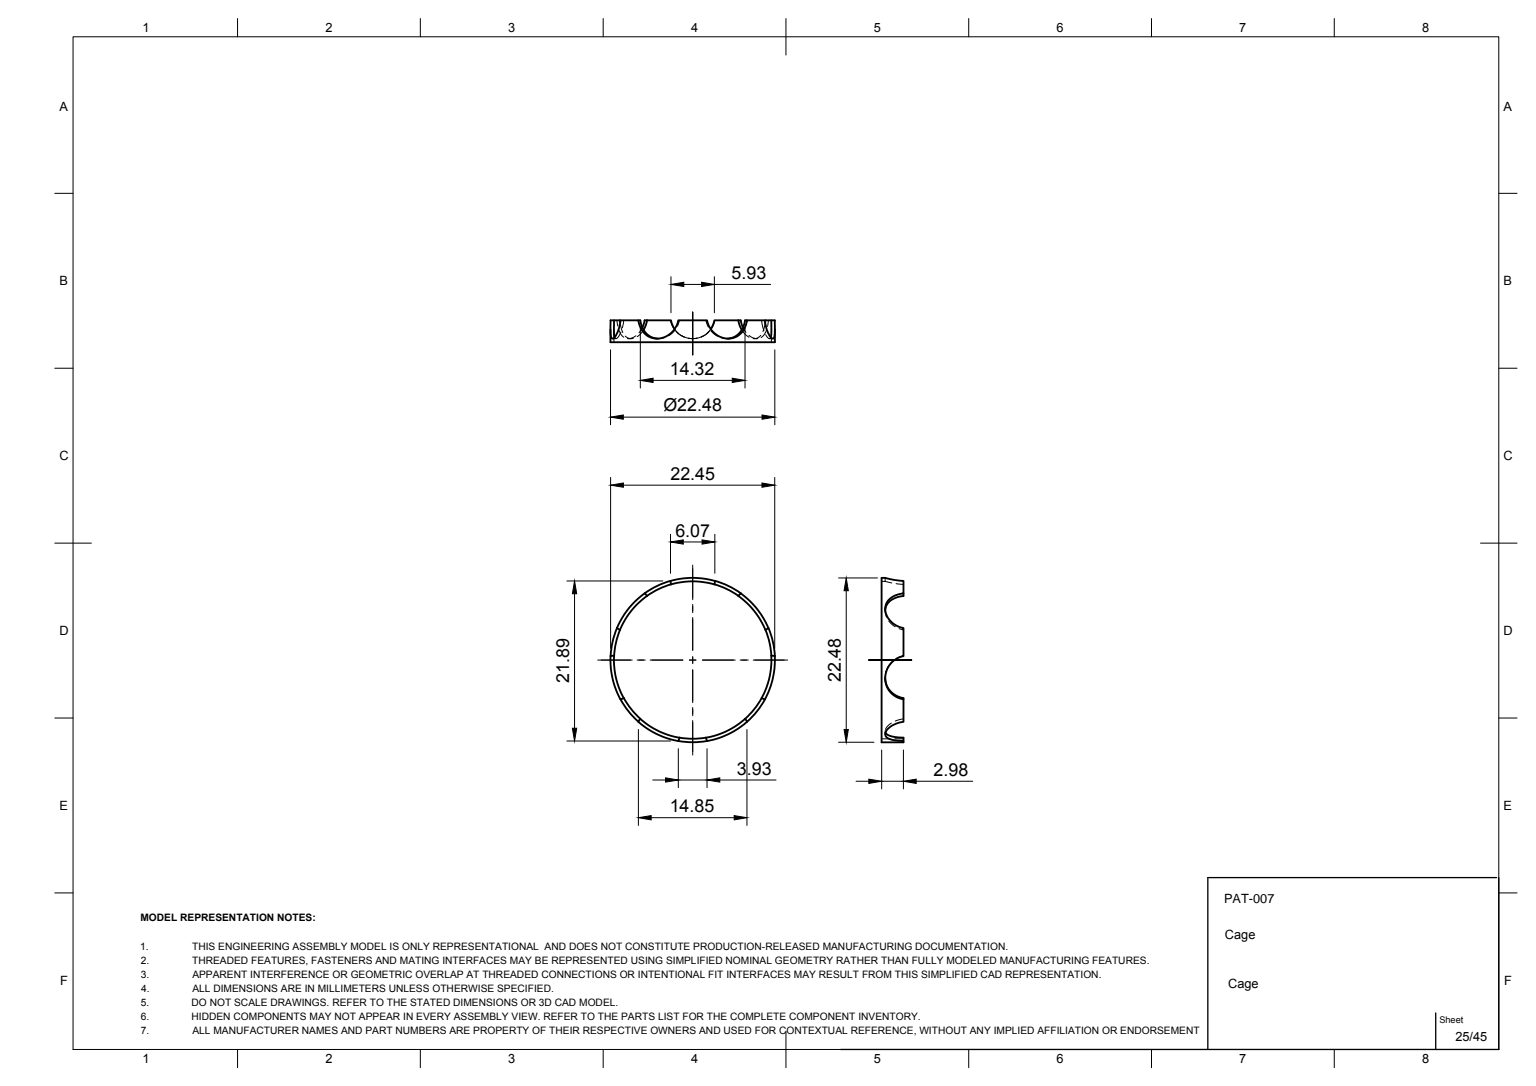
ISO-10303-21;
HEADER;
/* Generated by software containing ST-Developer
 * from STEP Tools, Inc. (www.steptools.com) 
 */

FILE_DESCRIPTION(
/* description */ ('Bearing friction torque test rig'),
/* implementation_level */ '2;1');

FILE_NAME(
/* name */ 'Cage.step',
/* time_stamp */ '2026-10-28T03:24:04-07:00',
/* author */ (''),
/* organization */ (''),
/* preprocessor_version */ 'ST-DEVELOPER v20.2',
/* originating_system */ 'Autodesk Translation Framework v15.17.0.0',
/* authorisation */ '');

FILE_SCHEMA (('AUTOMOTIVE_DESIGN { 1 0 10303 214 3 1 1 }'));
ENDSEC;

DATA;
#10=MECHANICAL_DESIGN_GEOMETRIC_PRESENTATION_REPRESENTATION('',(#564),#14822);
#343=B_SPLINE_CURVE_WITH_KNOTS('',3,(#12896,#12897,#12898,#12899,#12900,
#12901,#12902,#12903,#12904,#12905,#12906,#12907,#12908,#12909,#12910,#12911,
#12912,#12913,#12914,#12915,#12916,#12917),.UNSPECIFIED.,.F.,.F.,(4,2,2,
2,2,2,2,2,2,2,4),(0.0591825211272536,0.157966726598481,0.236950089897721,
0.315933453196962,0.391576304923761,0.46721915665056,0.54286200837736,0.618504860104159,
0.697488223403399,0.77647158670264,0.875255792173867),.UNSPECIFIED.);
#344=B_SPLINE_CURVE_WITH_KNOTS('',3,(#12921,#12922,#12923,#12924,#12925,
#12926,#12927,#12928,#12929,#12930,#12931,#12932,#12933,#12934,#12935,#12936,
#12937,#12938,#12939,#12940,#12941,#12942),.UNSPECIFIED.,.F.,.F.,(4,2,2,
2,2,2,2,2,2,2,4),(0.0581119756758434,0.106553146291161,0.213106292582322,
0.30849933801665,0.386091982889075,0.4636846277615,0.541277272633925,0.61886991750635,
0.714262962940678,0.820816109231839,0.869257279847157),.UNSPECIFIED.);
#345=B_SPLINE_CURVE_WITH_KNOTS('',3,(#12948,#12949,#12950,#12951,#12952,
#12953,#12954,#12955,#12956,#12957,#12958,#12959,#12960,#12961,#12962,#12963,
#12964,#12965,#12966,#12967,#12968,#12969),.UNSPECIFIED.,.F.,.F.,(4,2,2,
2,2,2,2,2,2,2,4),(0.0581119756758434,0.106553146291161,0.213106292582322,
0.30849933801665,0.386091982889075,0.4636846277615,0.541277272633925,0.61886991750635,
0.714262962940679,0.820816109231839,0.869257279847157),.UNSPECIFIED.);
#346=B_SPLINE_CURVE_WITH_KNOTS('',3,(#12973,#12974,#12975,#12976,#12977,
#12978,#12979,#12980,#12981,#12982,#12983,#12984,#12985,#12986,#12987,#12988,
#12989,#12990,#12991,#12992,#12993,#12994),.UNSPECIFIED.,.F.,.F.,(4,2,2,
2,2,2,2,2,2,2,4),(0.0581119756758433,0.106553146291161,0.213106292582322,
0.308499338016649,0.386091982889075,0.4636846277615,0.541277272633925,0.61886991750635,
0.714262962940678,0.820816109231839,0.869257279847157),.UNSPECIFIED.);
#347=B_SPLINE_CURVE_WITH_KNOTS('',3,(#13003,#13004,#13005,#13006,#13007,
#13008,#13009,#13010,#13011,#13012,#13013,#13014,#13015,#13016,#13017,#13018,
#13019,#13020,#13021,#13022,#13023,#13024),.UNSPECIFIED.,.F.,.F.,(4,2,2,
2,2,2,2,2,2,2,4),(0.0581119756758433,0.106553146291161,0.213106292582322,
0.30849933801665,0.386091982889075,0.4636846277615,0.541277272633925,0.61886991750635,
0.714262962940678,0.820816109231839,0.869257279847157),.UNSPECIFIED.);
#348=B_SPLINE_CURVE_WITH_KNOTS('',3,(#13028,#13029,#13030,#13031,#13032,
#13033,#13034,#13035,#13036,#13037,#13038,#13039,#13040,#13041,#13042,#13043,
#13044,#13045,#13046,#13047,#13048,#13049),.UNSPECIFIED.,.F.,.F.,(4,2,2,
2,2,2,2,2,2,2,4),(0.0581119756758434,0.106553146291161,0.213106292582322,
0.30849933801665,0.386091982889075,0.4636846277615,0.541277272633925,0.61886991750635,
0.714262962940678,0.820816109231839,0.869257279847157),.UNSPECIFIED.);
#349=B_SPLINE_CURVE_WITH_KNOTS('',3,(#13053,#13054,#13055,#13056,#13057,
#13058,#13059,#13060,#13061,#13062,#13063,#13064,#13065,#13066,#13067,#13068,
#13069,#13070,#13071,#13072,#13073,#13074),.UNSPECIFIED.,.F.,.F.,(4,2,2,
2,2,2,2,2,2,2,4),(0.0581119756758434,0.106553146291161,0.213106292582322,
0.30849933801665,0.386091982889075,0.4636846277615,0.541277272633925,0.61886991750635,
0.714262962940678,0.820816109231839,0.869257279847157),.UNSPECIFIED.);
#350=B_SPLINE_CURVE_WITH_KNOTS('',3,(#13078,#13079,#13080,#13081,#13082,
#13083,#13084,#13085,#13086,#13087,#13088,#13089,#13090,#13091,#13092,#13093,
#13094,#13095,#13096,#13097,#13098,#13099),.UNSPECIFIED.,.F.,.F.,(4,2,2,
2,2,2,2,2,2,2,4),(0.0581119756758433,0.106553146291161,0.213106292582322,
0.30849933801665,0.386091982889075,0.4636846277615,0.541277272633925,0.61886991750635,
0.714262962940678,0.820816109231839,0.869257279847157),.UNSPECIFIED.);
#351=B_SPLINE_CURVE_WITH_KNOTS('',3,(#13107,#13108,#13109,#13110,#13111,
#13112,#13113,#13114,#13115,#13116,#13117,#13118,#13119,#13120,#13121,#13122,
#13123,#13124,#13125,#13126,#13127,#13128),.UNSPECIFIED.,.F.,.F.,(4,2,2,
2,2,2,2,2,2,2,4),(0.0591825211272536,0.157966726598481,0.236950089897721,
0.315933453196962,0.391576304923761,0.467219156650561,0.54286200837736,
0.618504860104159,0.697488223403399,0.77647158670264,0.875255792173867),
 .UNSPECIFIED.);
#352=B_SPLINE_CURVE_WITH_KNOTS('',3,(#13136,#13137,#13138,#13139,#13140,
#13141,#13142,#13143,#13144,#13145,#13146,#13147,#13148,#13149,#13150,#13151,
#13152,#13153,#13154,#13155,#13156,#13157),.UNSPECIFIED.,.F.,.F.,(4,2,2,
2,2,2,2,2,2,2,4),(0.0591825211272536,0.157966726598481,0.236950089897722,
0.315933453196962,0.391576304923761,0.467219156650561,0.54286200837736,
0.618504860104159,0.697488223403399,0.77647158670264,0.875255792173867),
 .UNSPECIFIED.);
#353=B_SPLINE_CURVE_WITH_KNOTS('',3,(#13167,#13168,#13169,#13170,#13171,
#13172,#13173,#13174,#13175,#13176,#13177,#13178,#13179,#13180,#13181,#13182,
#13183,#13184,#13185,#13186,#13187,#13188),.UNSPECIFIED.,.F.,.F.,(4,2,2,
2,2,2,2,2,2,2,4),(0.0591825211272536,0.157966726598481,0.236950089897721,
0.315933453196962,0.391576304923761,0.46721915665056,0.54286200837736,0.618504860104159,
0.697488223403399,0.77647158670264,0.875255792173867),.UNSPECIFIED.);
#354=B_SPLINE_CURVE_WITH_KNOTS('',3,(#13196,#13197,#13198,#13199,#13200,
#13201,#13202,#13203,#13204,#13205,#13206,#13207,#13208,#13209,#13210,#13211,
#13212,#13213,#13214,#13215,#13216,#13217),.UNSPECIFIED.,.F.,.F.,(4,2,2,
2,2,2,2,2,2,2,4),(0.0591825211272536,0.157966726598481,0.236950089897721,
0.315933453196962,0.391576304923761,0.46721915665056,0.542862008377359,
0.618504860104159,0.697488223403399,0.776471586702639,0.875255792173867),
 .UNSPECIFIED.);
#355=B_SPLINE_CURVE_WITH_KNOTS('',3,(#13225,#13226,#13227,#13228,#13229,
#13230,#13231,#13232,#13233,#13234,#13235,#13236,#13237,#13238,#13239,#13240,
#13241,#13242,#13243,#13244,#13245,#13246),.UNSPECIFIED.,.F.,.F.,(4,2,2,
2,2,2,2,2,2,2,4),(0.0591825211272536,0.157966726598481,0.236950089897721,
0.315933453196962,0.391576304923761,0.46721915665056,0.54286200837736,0.618504860104159,
0.697488223403399,0.77647158670264,0.875255792173867),.UNSPECIFIED.);
#356=B_SPLINE_CURVE_WITH_KNOTS('',3,(#13255,#13256,#13257,#13258,#13259,
#13260,#13261,#13262,#13263,#13264,#13265,#13266,#13267,#13268,#13269,#13270,
#13271,#13272,#13273,#13274,#13275,#13276),.UNSPECIFIED.,.F.,.F.,(4,2,2,
2,2,2,2,2,2,2,4),(0.0591825211272536,0.157966726598481,0.236950089897721,
0.315933453196962,0.391576304923761,0.46721915665056,0.542862008377359,
0.618504860104159,0.697488223403399,0.776471586702639,0.875255792173867),
 .UNSPECIFIED.);
#402=SPHERICAL_SURFACE('',#8679,0.309556);
#403=SPHERICAL_SURFACE('',#8695,0.309556);
#404=SPHERICAL_SURFACE('',#8700,0.309556);
#405=SPHERICAL_SURFACE('',#8706,0.309556);
#406=SPHERICAL_SURFACE('',#8711,0.309556);
#407=SPHERICAL_SURFACE('',#8716,0.309556);
#408=SPHERICAL_SURFACE('',#8724,0.309556);
#480=SHAPE_REPRESENTATION_RELATIONSHIP('SRR','None',#15020,#519);
#519=ADVANCED_BREP_SHAPE_REPRESENTATION('',(#617),#14800);
#564=STYLED_ITEM('',(#15284),#617);
#617=MANIFOLD_SOLID_BREP('Continuous crown cage',#7681);
#818=FACE_BOUND('',#1994,.T.);
#1006=PLANE('',#8692);
#1007=PLANE('',#8697);
#1008=PLANE('',#8702);
#1009=PLANE('',#8708);
#1010=PLANE('',#8713);
#1011=PLANE('',#8722);
#1012=PLANE('',#8726);
#1013=PLANE('',#8727);
#1359=FACE_OUTER_BOUND('',#1978,.T.);
#1360=FACE_OUTER_BOUND('',#1979,.T.);
#1361=FACE_OUTER_BOUND('',#1980,.T.);
#1362=FACE_OUTER_BOUND('',#1981,.T.);
#1363=FACE_OUTER_BOUND('',#1982,.T.);
#1364=FACE_OUTER_BOUND('',#1983,.T.);
#1365=FACE_OUTER_BOUND('',#1984,.T.);
#1366=FACE_OUTER_BOUND('',#1985,.T.);
#1367=FACE_OUTER_BOUND('',#1986,.T.);
#1368=FACE_OUTER_BOUND('',#1987,.T.);
#1369=FACE_OUTER_BOUND('',#1988,.T.);
#1370=FACE_OUTER_BOUND('',#1989,.T.);
#1371=FACE_OUTER_BOUND('',#1990,.T.);
#1372=FACE_OUTER_BOUND('',#1991,.T.);
#1373=FACE_OUTER_BOUND('',#1992,.T.);
#1374=FACE_OUTER_BOUND('',#1993,.T.);
#1375=FACE_OUTER_BOUND('',#1995,.T.);
#1978=EDGE_LOOP('',(#6282,#6283,#6284,#6285));
#1979=EDGE_LOOP('',(#6286,#6287,#6288,#6289,#6290,#6291,#6292,#6293,#6294,
#6295,#6296,#6297,#6298,#6299,#6300,#6301,#6302,#6303));
#1980=EDGE_LOOP('',(#6304,#6305,#6306,#6307));
#1981=EDGE_LOOP('',(#6308,#6309,#6310,#6311));
#1982=EDGE_LOOP('',(#6312,#6313,#6314,#6315));
#1983=EDGE_LOOP('',(#6316,#6317,#6318,#6319));
#1984=EDGE_LOOP('',(#6320,#6321,#6322,#6323,#6324,#6325));
#1985=EDGE_LOOP('',(#6326,#6327,#6328,#6329));
#1986=EDGE_LOOP('',(#6330,#6331,#6332,#6333));
#1987=EDGE_LOOP('',(#6334,#6335,#6336,#6337));
#1988=EDGE_LOOP('',(#6338,#6339,#6340,#6341));
#1989=EDGE_LOOP('',(#6342,#6343,#6344,#6345));
#1990=EDGE_LOOP('',(#6346,#6347,#6348,#6349,#6350,#6351,#6352,#6353,#6354,
#6355,#6356,#6357,#6358,#6359,#6360,#6361,#6362,#6363));
#1991=EDGE_LOOP('',(#6364,#6365,#6366,#6367));
#1992=EDGE_LOOP('',(#6368,#6369,#6370,#6371));
#1993=EDGE_LOOP('',(#6372));
#1994=EDGE_LOOP('',(#6373));
#1995=EDGE_LOOP('',(#6374,#6375,#6376,#6377));
#2532=LINE('',#12998,#2976);
#2533=LINE('',#13251,#2977);
#2976=VECTOR('',#10567,1.123812);
#2977=VECTOR('',#10636,1.076188);
#3355=CIRCLE('',#8680,0.303778037777585);
#3356=CIRCLE('',#8681,0.303778037777585);
#3357=CIRCLE('',#8683,1.123812);
#3358=CIRCLE('',#8684,1.123812);
#3359=CIRCLE('',#8685,1.123812);
#3360=CIRCLE('',#8686,1.123812);
#3361=CIRCLE('',#8687,1.123812);
#3362=CIRCLE('',#8688,1.123812);
#3363=CIRCLE('',#8689,1.123812);
#3364=CIRCLE('',#8690,1.123812);
#3365=CIRCLE('',#8691,1.123812);
#3366=CIRCLE('',#8693,1.076188);
#3367=CIRCLE('',#8694,0.303778037777585);
#3368=CIRCLE('',#8696,0.303778037777585);
#3369=CIRCLE('',#8698,1.076188);
#3370=CIRCLE('',#8699,0.303778037777585);
#3371=CIRCLE('',#8701,0.303778037777585);
#3372=CIRCLE('',#8703,1.076188);
#3373=CIRCLE('',#8704,1.076188);
#3374=CIRCLE('',#8705,0.303778037777585);
#3375=CIRCLE('',#8707,0.303778037777585);
#3376=CIRCLE('',#8709,1.076188);
#3377=CIRCLE('',#8710,0.303778037777585);
#3378=CIRCLE('',#8712,0.303778037777585);
#3379=CIRCLE('',#8714,1.076188);
#3380=CIRCLE('',#8715,0.303778037777585);
#3381=CIRCLE('',#8717,0.303778037777585);
#3382=CIRCLE('',#8719,1.076188);
#3383=CIRCLE('',#8720,1.076188);
#3384=CIRCLE('',#8721,1.076188);
#3385=CIRCLE('',#8723,0.303778037777585);
#3386=CIRCLE('',#8725,0.303778037777585);
#3938=VERTEX_POINT('',#12894);
#3939=VERTEX_POINT('',#12895);
#3940=VERTEX_POINT('',#12918);
#3941=VERTEX_POINT('',#12920);
#3942=VERTEX_POINT('',#12945);
#3943=VERTEX_POINT('',#12947);
#3944=VERTEX_POINT('',#12970);
#3945=VERTEX_POINT('',#12972);
#3946=VERTEX_POINT('',#12995);
#3947=VERTEX_POINT('',#12997);
#3948=VERTEX_POINT('',#13000);
#3949=VERTEX_POINT('',#13002);
#3950=VERTEX_POINT('',#13025);
#3951=VERTEX_POINT('',#13027);
#3952=VERTEX_POINT('',#13050);
#3953=VERTEX_POINT('',#13052);
#3954=VERTEX_POINT('',#13075);
#3955=VERTEX_POINT('',#13077);
#3956=VERTEX_POINT('',#13102);
#3957=VERTEX_POINT('',#13106);
#3958=VERTEX_POINT('',#13131);
#3959=VERTEX_POINT('',#13135);
#3960=VERTEX_POINT('',#13160);
#3961=VERTEX_POINT('',#13162);
#3962=VERTEX_POINT('',#13166);
#3963=VERTEX_POINT('',#13191);
#3964=VERTEX_POINT('',#13195);
#3965=VERTEX_POINT('',#13220);
#3966=VERTEX_POINT('',#13224);
#3967=VERTEX_POINT('',#13249);
#3968=VERTEX_POINT('',#13252);
#3969=VERTEX_POINT('',#13254);
#4767=EDGE_CURVE('',#3938,#3939,#343,.T.);
#4768=EDGE_CURVE('',#3940,#3938,#3355,.T.);
#4769=EDGE_CURVE('',#3941,#3940,#344,.T.);
#4770=EDGE_CURVE('',#3939,#3941,#3356,.T.);
#4771=EDGE_CURVE('',#3942,#3940,#3357,.T.);
#4772=EDGE_CURVE('',#3942,#3943,#345,.T.);
#4773=EDGE_CURVE('',#3944,#3943,#3358,.T.);
#4774=EDGE_CURVE('',#3944,#3945,#346,.T.);
#4775=EDGE_CURVE('',#3946,#3945,#3359,.T.);
#4776=EDGE_CURVE('',#3946,#3947,#2532,.T.);
#4777=EDGE_CURVE('',#3947,#3947,#3360,.T.);
#4778=EDGE_CURVE('',#3948,#3946,#3361,.T.);
#4779=EDGE_CURVE('',#3948,#3949,#347,.T.);
#4780=EDGE_CURVE('',#3950,#3949,#3362,.T.);
#4781=EDGE_CURVE('',#3950,#3951,#348,.T.);
#4782=EDGE_CURVE('',#3952,#3951,#3363,.T.);
#4783=EDGE_CURVE('',#3952,#3953,#349,.T.);
#4784=EDGE_CURVE('',#3954,#3953,#3364,.T.);
#4785=EDGE_CURVE('',#3954,#3955,#350,.T.);
#4786=EDGE_CURVE('',#3941,#3955,#3365,.T.);
#4787=EDGE_CURVE('',#3938,#3956,#3366,.T.);
#4788=EDGE_CURVE('',#3956,#3942,#3367,.T.);
#4789=EDGE_CURVE('',#3957,#3956,#351,.T.);
#4790=EDGE_CURVE('',#3943,#3957,#3368,.T.);
#4791=EDGE_CURVE('',#3957,#3958,#3369,.T.);
#4792=EDGE_CURVE('',#3958,#3944,#3370,.T.);
#4793=EDGE_CURVE('',#3959,#3958,#352,.T.);
#4794=EDGE_CURVE('',#3945,#3959,#3371,.T.);
#4795=EDGE_CURVE('',#3959,#3960,#3372,.T.);
#4796=EDGE_CURVE('',#3960,#3961,#3373,.T.);
#4797=EDGE_CURVE('',#3961,#3948,#3374,.T.);
#4798=EDGE_CURVE('',#3962,#3961,#353,.T.);
#4799=EDGE_CURVE('',#3949,#3962,#3375,.T.);
#4800=EDGE_CURVE('',#3962,#3963,#3376,.T.);
#4801=EDGE_CURVE('',#3963,#3950,#3377,.T.);
#4802=EDGE_CURVE('',#3964,#3963,#354,.T.);
#4803=EDGE_CURVE('',#3951,#3964,#3378,.T.);
#4804=EDGE_CURVE('',#3964,#3965,#3379,.T.);
#4805=EDGE_CURVE('',#3965,#3952,#3380,.T.);
#4806=EDGE_CURVE('',#3966,#3965,#355,.T.);
#4807=EDGE_CURVE('',#3953,#3966,#3381,.T.);
#4808=EDGE_CURVE('',#3967,#3967,#3382,.T.);
#4809=EDGE_CURVE('',#3967,#3960,#2533,.T.);
#4810=EDGE_CURVE('',#3968,#3939,#3383,.T.);
#4811=EDGE_CURVE('',#3968,#3969,#356,.T.);
#4812=EDGE_CURVE('',#3966,#3969,#3384,.T.);
#4813=EDGE_CURVE('',#3955,#3968,#3385,.T.);
#4814=EDGE_CURVE('',#3969,#3954,#3386,.T.);
#6282=ORIENTED_EDGE('',*,*,#4767,.F.);
#6283=ORIENTED_EDGE('',*,*,#4768,.F.);
#6284=ORIENTED_EDGE('',*,*,#4769,.F.);
#6285=ORIENTED_EDGE('',*,*,#4770,.F.);
#6286=ORIENTED_EDGE('',*,*,#4769,.T.);
#6287=ORIENTED_EDGE('',*,*,#4771,.F.);
#6288=ORIENTED_EDGE('',*,*,#4772,.T.);
#6289=ORIENTED_EDGE('',*,*,#4773,.F.);
#6290=ORIENTED_EDGE('',*,*,#4774,.T.);
#6291=ORIENTED_EDGE('',*,*,#4775,.F.);
#6292=ORIENTED_EDGE('',*,*,#4776,.T.);
#6293=ORIENTED_EDGE('',*,*,#4777,.F.);
#6294=ORIENTED_EDGE('',*,*,#4776,.F.);
#6295=ORIENTED_EDGE('',*,*,#4778,.F.);
#6296=ORIENTED_EDGE('',*,*,#4779,.T.);
#6297=ORIENTED_EDGE('',*,*,#4780,.F.);
#6298=ORIENTED_EDGE('',*,*,#4781,.T.);
#6299=ORIENTED_EDGE('',*,*,#4782,.F.);
#6300=ORIENTED_EDGE('',*,*,#4783,.T.);
#6301=ORIENTED_EDGE('',*,*,#4784,.F.);
#6302=ORIENTED_EDGE('',*,*,#4785,.T.);
#6303=ORIENTED_EDGE('',*,*,#4786,.F.);
#6304=ORIENTED_EDGE('',*,*,#4768,.T.);
#6305=ORIENTED_EDGE('',*,*,#4787,.T.);
#6306=ORIENTED_EDGE('',*,*,#4788,.T.);
#6307=ORIENTED_EDGE('',*,*,#4771,.T.);
#6308=ORIENTED_EDGE('',*,*,#4789,.F.);
#6309=ORIENTED_EDGE('',*,*,#4790,.F.);
#6310=ORIENTED_EDGE('',*,*,#4772,.F.);
#6311=ORIENTED_EDGE('',*,*,#4788,.F.);
#6312=ORIENTED_EDGE('',*,*,#4790,.T.);
#6313=ORIENTED_EDGE('',*,*,#4791,.T.);
#6314=ORIENTED_EDGE('',*,*,#4792,.T.);
#6315=ORIENTED_EDGE('',*,*,#4773,.T.);
#6316=ORIENTED_EDGE('',*,*,#4793,.F.);
#6317=ORIENTED_EDGE('',*,*,#4794,.F.);
#6318=ORIENTED_EDGE('',*,*,#4774,.F.);
#6319=ORIENTED_EDGE('',*,*,#4792,.F.);
#6320=ORIENTED_EDGE('',*,*,#4794,.T.);
#6321=ORIENTED_EDGE('',*,*,#4795,.T.);
#6322=ORIENTED_EDGE('',*,*,#4796,.T.);
#6323=ORIENTED_EDGE('',*,*,#4797,.T.);
#6324=ORIENTED_EDGE('',*,*,#4778,.T.);
#6325=ORIENTED_EDGE('',*,*,#4775,.T.);
#6326=ORIENTED_EDGE('',*,*,#4798,.F.);
#6327=ORIENTED_EDGE('',*,*,#4799,.F.);
#6328=ORIENTED_EDGE('',*,*,#4779,.F.);
#6329=ORIENTED_EDGE('',*,*,#4797,.F.);
#6330=ORIENTED_EDGE('',*,*,#4799,.T.);
#6331=ORIENTED_EDGE('',*,*,#4800,.T.);
#6332=ORIENTED_EDGE('',*,*,#4801,.T.);
#6333=ORIENTED_EDGE('',*,*,#4780,.T.);
#6334=ORIENTED_EDGE('',*,*,#4802,.F.);
#6335=ORIENTED_EDGE('',*,*,#4803,.F.);
#6336=ORIENTED_EDGE('',*,*,#4781,.F.);
#6337=ORIENTED_EDGE('',*,*,#4801,.F.);
#6338=ORIENTED_EDGE('',*,*,#4803,.T.);
#6339=ORIENTED_EDGE('',*,*,#4804,.T.);
#6340=ORIENTED_EDGE('',*,*,#4805,.T.);
#6341=ORIENTED_EDGE('',*,*,#4782,.T.);
#6342=ORIENTED_EDGE('',*,*,#4783,.F.);
#6343=ORIENTED_EDGE('',*,*,#4805,.F.);
#6344=ORIENTED_EDGE('',*,*,#4806,.F.);
#6345=ORIENTED_EDGE('',*,*,#4807,.F.);
#6346=ORIENTED_EDGE('',*,*,#4808,.F.);
#6347=ORIENTED_EDGE('',*,*,#4809,.T.);
#6348=ORIENTED_EDGE('',*,*,#4795,.F.);
#6349=ORIENTED_EDGE('',*,*,#4793,.T.);
#6350=ORIENTED_EDGE('',*,*,#4791,.F.);
#6351=ORIENTED_EDGE('',*,*,#4789,.T.);
#6352=ORIENTED_EDGE('',*,*,#4787,.F.);
#6353=ORIENTED_EDGE('',*,*,#4767,.T.);
#6354=ORIENTED_EDGE('',*,*,#4810,.F.);
#6355=ORIENTED_EDGE('',*,*,#4811,.T.);
#6356=ORIENTED_EDGE('',*,*,#4812,.F.);
#6357=ORIENTED_EDGE('',*,*,#4806,.T.);
#6358=ORIENTED_EDGE('',*,*,#4804,.F.);
#6359=ORIENTED_EDGE('',*,*,#4802,.T.);
#6360=ORIENTED_EDGE('',*,*,#4800,.F.);
#6361=ORIENTED_EDGE('',*,*,#4798,.T.);
#6362=ORIENTED_EDGE('',*,*,#4796,.F.);
#6363=ORIENTED_EDGE('',*,*,#4809,.F.);
#6364=ORIENTED_EDGE('',*,*,#4770,.T.);
#6365=ORIENTED_EDGE('',*,*,#4786,.T.);
#6366=ORIENTED_EDGE('',*,*,#4813,.T.);
#6367=ORIENTED_EDGE('',*,*,#4810,.T.);
#6368=ORIENTED_EDGE('',*,*,#4785,.F.);
#6369=ORIENTED_EDGE('',*,*,#4814,.F.);
#6370=ORIENTED_EDGE('',*,*,#4811,.F.);
#6371=ORIENTED_EDGE('',*,*,#4813,.F.);
#6372=ORIENTED_EDGE('',*,*,#4777,.T.);
#6373=ORIENTED_EDGE('',*,*,#4808,.T.);
#6374=ORIENTED_EDGE('',*,*,#4807,.T.);
#6375=ORIENTED_EDGE('',*,*,#4812,.T.);
#6376=ORIENTED_EDGE('',*,*,#4814,.T.);
#6377=ORIENTED_EDGE('',*,*,#4784,.T.);
#7156=CYLINDRICAL_SURFACE('',#8682,1.123812);
#7157=CYLINDRICAL_SURFACE('',#8718,1.076188);
#7470=ADVANCED_FACE('',(#1359),#402,.F.);
#7471=ADVANCED_FACE('',(#1360),#7156,.T.);
#7472=ADVANCED_FACE('',(#1361),#1006,.T.);
#7473=ADVANCED_FACE('',(#1362),#403,.F.);
#7474=ADVANCED_FACE('',(#1363),#1007,.T.);
#7475=ADVANCED_FACE('',(#1364),#404,.F.);
#7476=ADVANCED_FACE('',(#1365),#1008,.T.);
#7477=ADVANCED_FACE('',(#1366),#405,.F.);
#7478=ADVANCED_FACE('',(#1367),#1009,.T.);
#7479=ADVANCED_FACE('',(#1368),#406,.F.);
#7480=ADVANCED_FACE('',(#1369),#1010,.T.);
#7481=ADVANCED_FACE('',(#1370),#407,.F.);
#7482=ADVANCED_FACE('',(#1371),#7157,.F.);
#7483=ADVANCED_FACE('',(#1372),#1011,.T.);
#7484=ADVANCED_FACE('',(#1373),#408,.F.);
#7485=ADVANCED_FACE('',(#1374,#818),#1012,.T.);
#7486=ADVANCED_FACE('',(#1375),#1013,.T.);
#7681=CLOSED_SHELL('',(#7470,#7471,#7472,#7473,#7474,#7475,#7476,#7477,
#7478,#7479,#7480,#7481,#7482,#7483,#7484,#7485,#7486));
#8678=AXIS2_PLACEMENT_3D('',#12892,#10551,#10552);
#8679=AXIS2_PLACEMENT_3D('',#12893,#10553,#10554);
#8680=AXIS2_PLACEMENT_3D('',#12919,#10555,#10556);
#8681=AXIS2_PLACEMENT_3D('',#12943,#10557,#10558);
#8682=AXIS2_PLACEMENT_3D('',#12944,#10559,#10560);
#8683=AXIS2_PLACEMENT_3D('',#12946,#10561,#10562);
#8684=AXIS2_PLACEMENT_3D('',#12971,#10563,#10564);
#8685=AXIS2_PLACEMENT_3D('',#12996,#10565,#10566);
#8686=AXIS2_PLACEMENT_3D('',#12999,#10568,#10569);
#8687=AXIS2_PLACEMENT_3D('',#13001,#10570,#10571);
#8688=AXIS2_PLACEMENT_3D('',#13026,#10572,#10573);
#8689=AXIS2_PLACEMENT_3D('',#13051,#10574,#10575);
#8690=AXIS2_PLACEMENT_3D('',#13076,#10576,#10577);
#8691=AXIS2_PLACEMENT_3D('',#13100,#10578,#10579);
#8692=AXIS2_PLACEMENT_3D('',#13101,#10580,#10581);
#8693=AXIS2_PLACEMENT_3D('',#13103,#10582,#10583);
#8694=AXIS2_PLACEMENT_3D('',#13104,#10584,#10585);
#8695=AXIS2_PLACEMENT_3D('',#13105,#10586,#10587);
#8696=AXIS2_PLACEMENT_3D('',#13129,#10588,#10589);
#8697=AXIS2_PLACEMENT_3D('',#13130,#10590,#10591);
#8698=AXIS2_PLACEMENT_3D('',#13132,#10592,#10593);
#8699=AXIS2_PLACEMENT_3D('',#13133,#10594,#10595);
#8700=AXIS2_PLACEMENT_3D('',#13134,#10596,#10597);
#8701=AXIS2_PLACEMENT_3D('',#13158,#10598,#10599);
#8702=AXIS2_PLACEMENT_3D('',#13159,#10600,#10601);
#8703=AXIS2_PLACEMENT_3D('',#13161,#10602,#10603);
#8704=AXIS2_PLACEMENT_3D('',#13163,#10604,#10605);
#8705=AXIS2_PLACEMENT_3D('',#13164,#10606,#10607);
#8706=AXIS2_PLACEMENT_3D('',#13165,#10608,#10609);
#8707=AXIS2_PLACEMENT_3D('',#13189,#10610,#10611);
#8708=AXIS2_PLACEMENT_3D('',#13190,#10612,#10613);
#8709=AXIS2_PLACEMENT_3D('',#13192,#10614,#10615);
#8710=AXIS2_PLACEMENT_3D('',#13193,#10616,#10617);
#8711=AXIS2_PLACEMENT_3D('',#13194,#10618,#10619);
#8712=AXIS2_PLACEMENT_3D('',#13218,#10620,#10621);
#8713=AXIS2_PLACEMENT_3D('',#13219,#10622,#10623);
#8714=AXIS2_PLACEMENT_3D('',#13221,#10624,#10625);
#8715=AXIS2_PLACEMENT_3D('',#13222,#10626,#10627);
#8716=AXIS2_PLACEMENT_3D('',#13223,#10628,#10629);
#8717=AXIS2_PLACEMENT_3D('',#13247,#10630,#10631);
#8718=AXIS2_PLACEMENT_3D('',#13248,#10632,#10633);
#8719=AXIS2_PLACEMENT_3D('',#13250,#10634,#10635);
#8720=AXIS2_PLACEMENT_3D('',#13253,#10637,#10638);
#8721=AXIS2_PLACEMENT_3D('',#13277,#10639,#10640);
#8722=AXIS2_PLACEMENT_3D('',#13278,#10641,#10642);
#8723=AXIS2_PLACEMENT_3D('',#13279,#10643,#10644);
#8724=AXIS2_PLACEMENT_3D('',#13280,#10645,#10646);
#8725=AXIS2_PLACEMENT_3D('',#13281,#10647,#10648);
#8726=AXIS2_PLACEMENT_3D('',#13282,#10649,#10650);
#8727=AXIS2_PLACEMENT_3D('',#13283,#10651,#10652);
#10551=DIRECTION('axis',(0.,0.,1.));
#10552=DIRECTION('refdir',(1.,0.,0.));
#10553=DIRECTION('center_axis',(0.,0.,1.));
#10554=DIRECTION('ref_axis',(1.,0.,0.));
#10555=DIRECTION('center_axis',(0.,-1.,0.));
#10556=DIRECTION('ref_axis',(0.,0.,-1.));
#10557=DIRECTION('center_axis',(0.,-1.,0.));
#10558=DIRECTION('ref_axis',(0.,0.,-1.));
#10559=DIRECTION('center_axis',(0.,1.,0.));
#10560=DIRECTION('ref_axis',(1.,0.,0.));
#10561=DIRECTION('center_axis',(0.,1.,0.));
#10562=DIRECTION('ref_axis',(1.,0.,0.));
#10563=DIRECTION('center_axis',(0.,1.,0.));
#10564=DIRECTION('ref_axis',(1.,0.,0.));
#10565=DIRECTION('center_axis',(0.,1.,0.));
#10566=DIRECTION('ref_axis',(1.,0.,0.));
#10567=DIRECTION('',(0.,-1.,0.));
#10568=DIRECTION('center_axis',(0.,-1.,0.));
#10569=DIRECTION('ref_axis',(1.,0.,0.));
#10570=DIRECTION('center_axis',(0.,1.,0.));
#10571=DIRECTION('ref_axis',(1.,0.,0.));
#10572=DIRECTION('center_axis',(0.,1.,0.));
#10573=DIRECTION('ref_axis',(1.,0.,0.));
#10574=DIRECTION('center_axis',(0.,1.,0.));
#10575=DIRECTION('ref_axis',(1.,0.,0.));
#10576=DIRECTION('center_axis',(0.,1.,0.));
#10577=DIRECTION('ref_axis',(1.,0.,0.));
#10578=DIRECTION('center_axis',(0.,1.,0.));
#10579=DIRECTION('ref_axis',(1.,0.,0.));
#10580=DIRECTION('center_axis',(0.,1.,0.));
#10581=DIRECTION('ref_axis',(1.,0.,0.));
#10582=DIRECTION('center_axis',(0.,-1.,0.));
#10583=DIRECTION('ref_axis',(1.,0.,0.));
#10584=DIRECTION('center_axis',(0.,-1.,0.));
#10585=DIRECTION('ref_axis',(0.,0.,-1.));
#10586=DIRECTION('center_axis',(8.96625347776458E-17,0.,1.));
#10587=DIRECTION('ref_axis',(1.,0.,0.));
#10588=DIRECTION('center_axis',(0.,-1.,0.));
#10589=DIRECTION('ref_axis',(0.,0.,-1.));
#10590=DIRECTION('center_axis',(0.,1.,0.));
#10591=DIRECTION('ref_axis',(1.,0.,0.));
#10592=DIRECTION('center_axis',(0.,-1.,0.));
#10593=DIRECTION('ref_axis',(1.,0.,0.));
#10594=DIRECTION('center_axis',(0.,-1.,0.));
#10595=DIRECTION('ref_axis',(0.,0.,-1.));
#10596=DIRECTION('center_axis',(0.,0.,1.));
#10597=DIRECTION('ref_axis',(1.,0.,0.));
#10598=DIRECTION('center_axis',(0.,-1.,0.));
#10599=DIRECTION('ref_axis',(0.,0.,-1.));
#10600=DIRECTION('center_axis',(0.,1.,0.));
#10601=DIRECTION('ref_axis',(1.,0.,0.));
#10602=DIRECTION('center_axis',(0.,-1.,0.));
#10603=DIRECTION('ref_axis',(1.,0.,0.));
#10604=DIRECTION('center_axis',(0.,-1.,0.));
#10605=DIRECTION('ref_axis',(1.,0.,0.));
#10606=DIRECTION('center_axis',(0.,-1.,0.));
#10607=DIRECTION('ref_axis',(0.,0.,-1.));
#10608=DIRECTION('center_axis',(0.,0.,1.));
#10609=DIRECTION('ref_axis',(1.,0.,0.));
#10610=DIRECTION('center_axis',(0.,-1.,0.));
#10611=DIRECTION('ref_axis',(0.,0.,-1.));
#10612=DIRECTION('center_axis',(0.,1.,0.));
#10613=DIRECTION('ref_axis',(1.,0.,0.));
#10614=DIRECTION('center_axis',(0.,-1.,0.));
#10615=DIRECTION('ref_axis',(1.,0.,0.));
#10616=DIRECTION('center_axis',(0.,-1.,0.));
#10617=DIRECTION('ref_axis',(0.,0.,-1.));
#10618=DIRECTION('center_axis',(8.96625347776458E-17,0.,1.));
#10619=DIRECTION('ref_axis',(1.,0.,0.));
#10620=DIRECTION('center_axis',(0.,-1.,0.));
#10621=DIRECTION('ref_axis',(0.,0.,-1.));
#10622=DIRECTION('center_axis',(0.,1.,0.));
#10623=DIRECTION('ref_axis',(1.,0.,0.));
#10624=DIRECTION('center_axis',(0.,-1.,0.));
#10625=DIRECTION('ref_axis',(1.,0.,0.));
#10626=DIRECTION('center_axis',(0.,-1.,0.));
#10627=DIRECTION('ref_axis',(0.,0.,-1.));
#10628=DIRECTION('center_axis',(0.,0.,1.));
#10629=DIRECTION('ref_axis',(1.,0.,0.));
#10630=DIRECTION('center_axis',(0.,-1.,0.));
#10631=DIRECTION('ref_axis',(0.,0.,-1.));
#10632=DIRECTION('center_axis',(0.,1.,0.));
#10633=DIRECTION('ref_axis',(1.,0.,0.));
#10634=DIRECTION('center_axis',(0.,1.,0.));
#10635=DIRECTION('ref_axis',(1.,0.,0.));
#10636=DIRECTION('',(0.,1.,0.));
#10637=DIRECTION('center_axis',(0.,-1.,0.));
#10638=DIRECTION('ref_axis',(1.,0.,0.));
#10639=DIRECTION('center_axis',(0.,-1.,0.));
#10640=DIRECTION('ref_axis',(1.,0.,0.));
#10641=DIRECTION('center_axis',(0.,1.,0.));
#10642=DIRECTION('ref_axis',(1.,0.,0.));
#10643=DIRECTION('center_axis',(0.,-1.,0.));
#10644=DIRECTION('ref_axis',(0.,0.,-1.));
#10645=DIRECTION('center_axis',(0.,0.,1.));
#10646=DIRECTION('ref_axis',(1.,0.,0.));
#10647=DIRECTION('center_axis',(0.,-1.,0.));
#10648=DIRECTION('ref_axis',(0.,0.,-1.));
#10649=DIRECTION('center_axis',(0.,-1.,0.));
#10650=DIRECTION('ref_axis',(-1.,0.,0.));
#10651=DIRECTION('center_axis',(0.,1.,0.));
#10652=DIRECTION('ref_axis',(1.,0.,0.));
#12892=CARTESIAN_POINT('',(0.,0.,0.));
#12893=CARTESIAN_POINT('Origin',(0.685838782044607,0.,0.860014630714833));
#12894=CARTESIAN_POINT('',(0.413083465285518,-0.05953,0.993751811093549));
#12895=CARTESIAN_POINT('',(0.876916659919095,-0.05953,0.623857181492959));
#12896=CARTESIAN_POINT('Ctrl Pts',(0.413083465285518,-0.05953,0.993751811093549));
#12897=CARTESIAN_POINT('Ctrl Pts',(0.419070565453383,-0.0925528133349865,
0.991263089003441));
#12898=CARTESIAN_POINT('Ctrl Pts',(0.430199341854858,-0.124911173756694,
0.986608710139579));
#12899=CARTESIAN_POINT('Ctrl Pts',(0.457978755888596,-0.177924977804098,
0.973971221090534));
#12900=CARTESIAN_POINT('Ctrl Pts',(0.473077587363685,-0.199697230012983,
0.966820759530997));
#12901=CARTESIAN_POINT('Ctrl Pts',(0.507057380724533,-0.237895043532788,
0.949440676105255));
#12902=CARTESIAN_POINT('Ctrl Pts',(0.525933334162555,-0.254319232363049,
0.939198248544428));
#12903=CARTESIAN_POINT('Ctrl Pts',(0.564362943424238,-0.28018331644634,
0.916597376014514));
#12904=CARTESIAN_POINT('Ctrl Pts',(0.585840553788742,-0.29104845371857,
0.903141581680914));
#12905=CARTESIAN_POINT('Ctrl Pts',(0.629305439856167,-0.30527573347708,
0.873412008702649));
#12906=CARTESIAN_POINT('Ctrl Pts',(0.651278921914856,-0.308638795020976,
0.857118508332695));
#12907=CARTESIAN_POINT('Ctrl Pts',(0.690705563850638,-0.308638795020976,
0.825676810575914));
#12908=CARTESIAN_POINT('Ctrl Pts',(0.711480111898423,-0.30527573347708,
0.807879894508811));
#12909=CARTESIAN_POINT('Ctrl Pts',(0.750136149454208,-0.29104845371857,
0.772120216227122));
#12910=CARTESIAN_POINT('Ctrl Pts',(0.768033796848072,-0.28018331644634,
0.754175290318038));
#12911=CARTESIAN_POINT('Ctrl Pts',(0.798619410861634,-0.254319232363049,
0.721738358858166));
#12912=CARTESIAN_POINT('Ctrl Pts',(0.812805334167529,-0.237895043532788,
0.705614819529209));
#12913=CARTESIAN_POINT('Ctrl Pts',(0.837310877969633,-0.199697230012983,
0.676354402927683));
#12914=CARTESIAN_POINT('Ctrl Pts',(0.847641868610495,-0.177924977804098,
0.663225258065736));
#12915=CARTESIAN_POINT('Ctrl Pts',(0.866144010579847,-0.124911173756694,
0.638954437806245));
#12916=CARTESIAN_POINT('Ctrl Pts',(0.873158080166742,-0.0925528133349865,
0.62914037979579));
#12917=CARTESIAN_POINT('Ctrl Pts',(0.876916659919095,-0.05953,0.623857181492959));
#12918=CARTESIAN_POINT('',(0.437601487681057,-0.05953,1.03511272300331));
#12919=CARTESIAN_POINT('Origin',(0.685838782044607,-0.05953,0.860014630714833));
#12920=CARTESIAN_POINT('',(0.911784794170997,-0.05953,0.656964154625313));
#12921=CARTESIAN_POINT('Ctrl Pts',(0.911784794170998,-0.0595300000000001,
0.656964154625312));
#12922=CARTESIAN_POINT('Ctrl Pts',(0.909827729890942,-0.0762225747374255,
0.659680317203144));
#12923=CARTESIAN_POINT('Ctrl Pts',(0.907004864562642,-0.0928409665394228,
0.663576540841106));
#12924=CARTESIAN_POINT('Ctrl Pts',(0.895234408667242,-0.144299303100741,
0.679480524217551));
#12925=CARTESIAN_POINT('Ctrl Pts',(0.882797231409153,-0.177024326825049,
0.695831250979106));
#12926=CARTESIAN_POINT('Ctrl Pts',(0.854332839576145,-0.227269801620064,
0.73042219438957));
#12927=CARTESIAN_POINT('Ctrl Pts',(0.834863020612702,-0.251265615809407,
0.752807465209441));
#12928=CARTESIAN_POINT('Ctrl Pts',(0.800439809856111,-0.279889827963178,
0.789147407129766));
#12929=CARTESIAN_POINT('Ctrl Pts',(0.781998747691871,-0.290879136862659,
0.80756613568454));
#12930=CARTESIAN_POINT('Ctrl Pts',(0.742239891936898,-0.305251990234487,
0.844254137480382));
#12931=CARTESIAN_POINT('Ctrl Pts',(0.720906778729541,-0.308638795020976,
0.862505527716294));
#12932=CARTESIAN_POINT('Ctrl Pts',(0.680463863683392,-0.308638795020976,
0.894757676234429));
#12933=CARTESIAN_POINT('Ctrl Pts',(0.657923009631182,-0.305251990234488,
0.91149460735272));
#12934=CARTESIAN_POINT('Ctrl Pts',(0.613307674922609,-0.290879136862659,
0.942092777160053));
#12935=CARTESIAN_POINT('Ctrl Pts',(0.591247219971725,-0.279889827963178,
0.955972930713954));
#12936=CARTESIAN_POINT('Ctrl Pts',(0.548158511259202,-0.251265615809407,
0.981446681891443));
#12937=CARTESIAN_POINT('Ctrl Pts',(0.522002043615455,-0.227269801620063,
0.995447160474328));
#12938=CARTESIAN_POINT('Ctrl Pts',(0.481944444320713,-0.177024326825049,
1.01550068154148));
#12939=CARTESIAN_POINT('Ctrl Pts',(0.463236132117164,-0.14429930310074,
1.0239876538093));
#12940=CARTESIAN_POINT('Ctrl Pts',(0.445111721969657,-0.0928409665394226,
1.03192403056628));
#12941=CARTESIAN_POINT('Ctrl Pts',(0.440685038163619,-0.0762225747374254,
1.03380912944435));
#12942=CARTESIAN_POINT('Ctrl Pts',(0.437601487681056,-0.05953,1.03511272300331));
#12943=CARTESIAN_POINT('Origin',(0.685838782044607,-0.05953,0.860014630714833));
#12944=CARTESIAN_POINT('Origin',(0.,-0.208355,0.));
#12945=CARTESIAN_POINT('',(0.0548532617164168,-0.05953,1.12247250791415));
#12946=CARTESIAN_POINT('Origin',(0.,-0.05953,0.));
#12947=CARTESIAN_POINT('',(-0.536443649899848,-0.05953,0.987512846410683));
#12948=CARTESIAN_POINT('Ctrl Pts',(0.0548532617164173,-0.0595300000000001,
1.12247250791414));
#12949=CARTESIAN_POINT('Ctrl Pts',(0.05150947068137,-0.0762225747374254,
1.12263591311425));
#12950=CARTESIAN_POINT('Ctrl Pts',(0.0467032526342597,-0.0928409665394227,
1.12285816383385));
#12951=CARTESIAN_POINT('Ctrl Pts',(0.0269302585198975,-0.144299303100741,
1.12357162229597));
#12952=CARTESIAN_POINT('Ctrl Pts',(0.006392292392153,-0.177024326825049,
1.12404235695137));
#12953=CARTESIAN_POINT('Ctrl Pts',(-0.0383992541984087,-0.227269801620063,
1.12335509974011));
#12954=CARTESIAN_POINT('Ctrl Pts',(-0.0680399972366993,-0.251265615809407,
1.12208997038458));
#12955=CARTESIAN_POINT('Ctrl Pts',(-0.117914228755037,-0.279889827963178,
1.1178344036749));
#12956=CARTESIAN_POINT('Ctrl Pts',(-0.14381238480104,-0.290879136862659,
1.11490049012186));
#12957=CARTESIAN_POINT('Ctrl Pts',(-0.19728546073067,-0.305251990234488,
1.10669035995599));
#12958=CARTESIAN_POINT('Ctrl Pts',(-0.224855950742601,-0.308638795020976,
1.10139101611326));
#12959=CARTESIAN_POINT('Ctrl Pts',(-0.275287440920027,-0.308638795020976,
1.0898803575765));
#12960=CARTESIAN_POINT('Ctrl Pts',(-0.302426893214945,-0.305251990234488,
1.08269251410343));
#12961=CARTESIAN_POINT('Ctrl Pts',(-0.35416671187353,-0.290879136862659,
1.06688848765783));
#12962=CARTESIAN_POINT('Ctrl Pts',(-0.3787731215897,-0.279889827963178,
1.05829506364875));
#12963=CARTESIAN_POINT('Ctrl Pts',(-0.425554672694338,-0.251265615809407,
1.04048957871266));
#12964=CARTESIAN_POINT('Ctrl Pts',(-0.452808978448581,-0.227269801620063,
1.02876878445619));
#12965=CARTESIAN_POINT('Ctrl Pts',(-0.493462957200432,-0.177024326825049,
1.0099536580922));
#12966=CARTESIAN_POINT('Ctrl Pts',(-0.511762781179148,-0.14429930310074,
1.00061845128527));
#12967=CARTESIAN_POINT('Ctrl Pts',(-0.529268075276157,-0.0928409665394226,
0.991396466802468));
#12968=CARTESIAN_POINT('Ctrl Pts',(-0.533501897135713,-0.0762225747374254,
0.989110885965947));
#12969=CARTESIAN_POINT('Ctrl Pts',(-0.536443649899848,-0.0595300000000001,
0.987512846410683));
#12970=CARTESIAN_POINT('',(-0.843383895613249,-0.05953,0.742736168477219));
#12971=CARTESIAN_POINT('Origin',(0.,-0.05953,0.));
#12972=CARTESIAN_POINT('',(-1.10653577764992,-0.05953,0.196295654879792));
#12973=CARTESIAN_POINT('Ctrl Pts',(-0.843383895613249,-0.0595300000000001,
0.742736168477219));
#12974=CARTESIAN_POINT('Ctrl Pts',(-0.84559647055299,-0.0762225747374255,
0.740223768851062));
#12975=CARTESIAN_POINT('Ctrl Pts',(-0.848766861100456,-0.0928409665394227,
0.736604687327351));
#12976=CARTESIAN_POINT('Ctrl Pts',(-0.861652925570091,-0.144299303100741,
0.721590372101268));
#12977=CARTESIAN_POINT('Ctrl Pts',(-0.87482617317514,-0.177024326825049,
0.705826641853758));
#12978=CARTESIAN_POINT('Ctrl Pts',(-0.902215926359523,-0.227269801620063,
0.670378702718353));
#12979=CARTESIAN_POINT('Ctrl Pts',(-0.919707509403859,-0.251265615809407,
0.646415841396062));
#12980=CARTESIAN_POINT('Ctrl Pts',(-0.947476448101718,-0.279889827963178,
0.604769294586516));
#12981=CARTESIAN_POINT('Ctrl Pts',(-0.961329858300736,-0.290879136862659,
0.582692035672022));
#12982=CARTESIAN_POINT('Ctrl Pts',(-0.988250837578047,-0.305251990234488,
0.535766169015486));
#12983=CARTESIAN_POINT('Ctrl Pts',(-1.00129756308006,-0.308638795020976,
0.510906605094603));
#12984=CARTESIAN_POINT('Ctrl Pts',(-1.02374168767024,-0.308638795020976,
0.46430090015576));
#12985=CARTESIAN_POINT('Ctrl Pts',(-1.03504317708586,-0.305251990234488,
0.438600874831839));
#12986=CARTESIAN_POINT('Ctrl Pts',(-1.05494634094458,-0.290879136862659,
0.388295406390235));
#12987=CARTESIAN_POINT('Ctrl Pts',(-1.06356957703048,-0.279889827963178,
0.363699428370917));
#12988=CARTESIAN_POINT('Ctrl Pts',(-1.0788165083757,-0.251265615809407,
0.316022600643821));
#12989=CARTESIAN_POINT('Ctrl Pts',(-1.08664560412098,-0.227269801620063,
0.287406530683752));
#12990=CARTESIAN_POINT('Ctrl Pts',(-1.09728268713976,-0.177024326825049,
0.243890930799337));
#12991=CARTESIAN_POINT('Ctrl Pts',(-1.10139388218929,-0.144299303100741,
0.22376314604679));
#12992=CARTESIAN_POINT('Ctrl Pts',(-1.10509821673782,-0.0928409665394227,
0.204327142733961));
#12993=CARTESIAN_POINT('Ctrl Pts',(-1.10595102243643,-0.0762225747374254,
0.199591971170104));
#12994=CARTESIAN_POINT('Ctrl Pts',(-1.10653577764992,-0.0595300000000001,
0.196295654879792));
#12995=CARTESIAN_POINT('',(-1.123812,-0.05953,1.37627276864339E-16));
#12996=CARTESIAN_POINT('Origin',(0.,-0.05953,0.));
#12997=CARTESIAN_POINT('',(-1.123812,-0.35718,1.37627276864339E-16));
#12998=CARTESIAN_POINT('',(-1.123812,-0.208355,1.37627276864339E-16));
#12999=CARTESIAN_POINT('Origin',(0.,-0.35718,0.));
#13000=CARTESIAN_POINT('',(-1.10653577764992,-0.05953,-0.196295654879793));
#13001=CARTESIAN_POINT('Origin',(0.,-0.05953,0.));
#13002=CARTESIAN_POINT('',(-0.843383895613249,-0.05953,-0.742736168477219));
#13003=CARTESIAN_POINT('Ctrl Pts',(-1.10653577764992,-0.0595300000000001,
-0.196295654879792));
#13004=CARTESIAN_POINT('Ctrl Pts',(-1.10595102243643,-0.0762225747374255,
-0.199591971170104));
#13005=CARTESIAN_POINT('Ctrl Pts',(-1.10509821673782,-0.0928409665394228,
-0.204327142733962));
#13006=CARTESIAN_POINT('Ctrl Pts',(-1.10139388218929,-0.144299303100741,
-0.22376314604679));
#13007=CARTESIAN_POINT('Ctrl Pts',(-1.09728268713976,-0.177024326825049,
-0.243890930799338));
#13008=CARTESIAN_POINT('Ctrl Pts',(-1.08664560412098,-0.227269801620063,
-0.287406530683753));
#13009=CARTESIAN_POINT('Ctrl Pts',(-1.0788165083757,-0.251265615809407,
-0.316022600643821));
#13010=CARTESIAN_POINT('Ctrl Pts',(-1.06356957703048,-0.279889827963178,
-0.363699428370918));
#13011=CARTESIAN_POINT('Ctrl Pts',(-1.05494634094458,-0.290879136862659,
-0.388295406390235));
#13012=CARTESIAN_POINT('Ctrl Pts',(-1.03504317708586,-0.305251990234488,
-0.438600874831839));
#13013=CARTESIAN_POINT('Ctrl Pts',(-1.02374168767024,-0.308638795020976,
-0.46430090015576));
#13014=CARTESIAN_POINT('Ctrl Pts',(-1.00129756308006,-0.308638795020976,
-0.510906605094603));
#13015=CARTESIAN_POINT('Ctrl Pts',(-0.988250837578047,-0.305251990234488,
-0.535766169015486));
#13016=CARTESIAN_POINT('Ctrl Pts',(-0.961329858300736,-0.290879136862659,
-0.582692035672022));
#13017=CARTESIAN_POINT('Ctrl Pts',(-0.947476448101718,-0.279889827963178,
-0.604769294586516));
#13018=CARTESIAN_POINT('Ctrl Pts',(-0.919707509403859,-0.251265615809407,
-0.646415841396062));
#13019=CARTESIAN_POINT('Ctrl Pts',(-0.902215926359523,-0.227269801620064,
-0.670378702718353));
#13020=CARTESIAN_POINT('Ctrl Pts',(-0.87482617317514,-0.177024326825049,
-0.705826641853758));
#13021=CARTESIAN_POINT('Ctrl Pts',(-0.861652925570091,-0.144299303100741,
-0.721590372101268));
#13022=CARTESIAN_POINT('Ctrl Pts',(-0.848766861100456,-0.0928409665394229,
-0.736604687327351));
#13023=CARTESIAN_POINT('Ctrl Pts',(-0.84559647055299,-0.0762225747374255,
-0.740223768851063));
#13024=CARTESIAN_POINT('Ctrl Pts',(-0.843383895613249,-0.0595300000000001,
-0.742736168477219));
#13025=CARTESIAN_POINT('',(-0.536443649899847,-0.05953,-0.987512846410683));
#13026=CARTESIAN_POINT('Origin',(0.,-0.05953,0.));
#13027=CARTESIAN_POINT('',(0.0548532617164172,-0.05953,-1.12247250791415));
#13028=CARTESIAN_POINT('Ctrl Pts',(-0.536443649899848,-0.0595300000000001,
-0.987512846410683));
#13029=CARTESIAN_POINT('Ctrl Pts',(-0.533501897135712,-0.0762225747374254,
-0.989110885965947));
#13030=CARTESIAN_POINT('Ctrl Pts',(-0.529268075276156,-0.0928409665394227,
-0.991396466802469));
#13031=CARTESIAN_POINT('Ctrl Pts',(-0.511762781179147,-0.144299303100741,
-1.00061845128527));
#13032=CARTESIAN_POINT('Ctrl Pts',(-0.493462957200432,-0.177024326825049,
-1.0099536580922));
#13033=CARTESIAN_POINT('Ctrl Pts',(-0.45280897844858,-0.227269801620063,
-1.02876878445619));
#13034=CARTESIAN_POINT('Ctrl Pts',(-0.425554672694337,-0.251265615809407,
-1.04048957871266));
#13035=CARTESIAN_POINT('Ctrl Pts',(-0.3787731215897,-0.279889827963178,
-1.05829506364875));
#13036=CARTESIAN_POINT('Ctrl Pts',(-0.354166711873529,-0.290879136862659,
-1.06688848765783));
#13037=CARTESIAN_POINT('Ctrl Pts',(-0.302426893214944,-0.305251990234488,
-1.08269251410343));
#13038=CARTESIAN_POINT('Ctrl Pts',(-0.275287440920027,-0.308638795020976,
-1.0898803575765));
#13039=CARTESIAN_POINT('Ctrl Pts',(-0.224855950742601,-0.308638795020976,
-1.10139101611326));
#13040=CARTESIAN_POINT('Ctrl Pts',(-0.19728546073067,-0.305251990234488,
-1.10669035995599));
#13041=CARTESIAN_POINT('Ctrl Pts',(-0.143812384801039,-0.290879136862659,
-1.11490049012186));
#13042=CARTESIAN_POINT('Ctrl Pts',(-0.117914228755037,-0.279889827963178,
-1.1178344036749));
#13043=CARTESIAN_POINT('Ctrl Pts',(-0.0680399972366989,-0.251265615809407,
-1.12208997038458));
#13044=CARTESIAN_POINT('Ctrl Pts',(-0.0383992541984084,-0.227269801620063,
-1.12335509974011));
#13045=CARTESIAN_POINT('Ctrl Pts',(0.00639229239215326,-0.177024326825049,
-1.12404235695137));
#13046=CARTESIAN_POINT('Ctrl Pts',(0.0269302585198977,-0.144299303100741,
-1.12357162229597));
#13047=CARTESIAN_POINT('Ctrl Pts',(0.04670325263426,-0.0928409665394228,
-1.12285816383385));
#13048=CARTESIAN_POINT('Ctrl Pts',(0.0515094706813703,-0.0762225747374255,
-1.12263591311425));
#13049=CARTESIAN_POINT('Ctrl Pts',(0.0548532617164176,-0.0595300000000001,
-1.12247250791414));
#13050=CARTESIAN_POINT('',(0.437601487681057,-0.05953,-1.03511272300331));
#13051=CARTESIAN_POINT('Origin',(0.,-0.05953,0.));
#13052=CARTESIAN_POINT('',(0.911784794170997,-0.05953,-0.656964154625313));
#13053=CARTESIAN_POINT('Ctrl Pts',(0.437601487681056,-0.0595300000000001,
-1.03511272300331));
#13054=CARTESIAN_POINT('Ctrl Pts',(0.440685038163619,-0.0762225747374255,
-1.03380912944435));
#13055=CARTESIAN_POINT('Ctrl Pts',(0.445111721969657,-0.0928409665394228,
-1.03192403056628));
#13056=CARTESIAN_POINT('Ctrl Pts',(0.463236132117164,-0.144299303100741,
-1.0239876538093));
#13057=CARTESIAN_POINT('Ctrl Pts',(0.481944444320713,-0.177024326825049,
-1.01550068154148));
#13058=CARTESIAN_POINT('Ctrl Pts',(0.522002043615455,-0.227269801620064,
-0.995447160474328));
#13059=CARTESIAN_POINT('Ctrl Pts',(0.548158511259203,-0.251265615809407,
-0.981446681891443));
#13060=CARTESIAN_POINT('Ctrl Pts',(0.591247219971725,-0.279889827963178,
-0.955972930713954));
#13061=CARTESIAN_POINT('Ctrl Pts',(0.613307674922609,-0.290879136862659,
-0.942092777160053));
#13062=CARTESIAN_POINT('Ctrl Pts',(0.657923009631182,-0.305251990234487,
-0.91149460735272));
#13063=CARTESIAN_POINT('Ctrl Pts',(0.680463863683393,-0.308638795020976,
-0.894757676234429));
#13064=CARTESIAN_POINT('Ctrl Pts',(0.720906778729542,-0.308638795020976,
-0.862505527716294));
#13065=CARTESIAN_POINT('Ctrl Pts',(0.742239891936899,-0.305251990234488,
-0.844254137480381));
#13066=CARTESIAN_POINT('Ctrl Pts',(0.781998747691872,-0.290879136862659,
-0.80756613568454));
#13067=CARTESIAN_POINT('Ctrl Pts',(0.800439809856112,-0.279889827963178,
-0.789147407129765));
#13068=CARTESIAN_POINT('Ctrl Pts',(0.834863020612702,-0.251265615809407,
-0.752807465209441));
#13069=CARTESIAN_POINT('Ctrl Pts',(0.854332839576145,-0.227269801620064,
-0.73042219438957));
#13070=CARTESIAN_POINT('Ctrl Pts',(0.882797231409153,-0.177024326825049,
-0.695831250979106));
#13071=CARTESIAN_POINT('Ctrl Pts',(0.895234408667242,-0.144299303100741,
-0.679480524217551));
#13072=CARTESIAN_POINT('Ctrl Pts',(0.907004864562642,-0.0928409665394228,
-0.663576540841106));
#13073=CARTESIAN_POINT('Ctrl Pts',(0.909827729890942,-0.0762225747374256,
-0.659680317203144));
#13074=CARTESIAN_POINT('Ctrl Pts',(0.911784794170998,-0.0595300000000001,
-0.656964154625312));
#13075=CARTESIAN_POINT('',(1.08212377959455,-0.05953,-0.303251606722892));
#13076=CARTESIAN_POINT('Origin',(0.,-0.05953,0.));
#13077=CARTESIAN_POINT('',(1.08212377959455,-0.05953,0.303251606722892));
#13078=CARTESIAN_POINT('Ctrl Pts',(1.08212377959455,-0.0595300000000001,
-0.303251606722892));
#13079=CARTESIAN_POINT('Ctrl Pts',(1.0830271513892,-0.0762225747374255,
-0.300028012588062));
#13080=CARTESIAN_POINT('Ctrl Pts',(1.08431331394788,-0.0928409665394228,
-0.2953917518996));
#13081=CARTESIAN_POINT('Ctrl Pts',(1.08940878963422,-0.144299303100741,
-0.276273267473431));
#13082=CARTESIAN_POINT('Ctrl Pts',(1.09443784939331,-0.177024326825049,
-0.256354979351213));
#13083=CARTESIAN_POINT('Ctrl Pts',(1.10373487993589,-0.227269801620064,
-0.212533521233765));
#13084=CARTESIAN_POINT('Ctrl Pts',(1.10909715583869,-0.251265615809407,
-0.183354415742157));
#13085=CARTESIAN_POINT('Ctrl Pts',(1.1160463456491,-0.279889827963178,-0.133783682657561));
#13086=CARTESIAN_POINT('Ctrl Pts',(1.11894887330541,-0.290879136862659,
-0.107881990270302));
#13087=CARTESIAN_POINT('Ctrl Pts',(1.12284346704144,-0.305251990234488,
-0.0539226701638766));
#13088=CARTESIAN_POINT('Ctrl Pts',(1.123812,-0.308638795020976,-0.025864214957475));
#13089=CARTESIAN_POINT('Ctrl Pts',(1.123812,-0.308638795020976,0.025864214957475));
#13090=CARTESIAN_POINT('Ctrl Pts',(1.12284346704144,-0.305251990234488,
0.0539226701638766));
#13091=CARTESIAN_POINT('Ctrl Pts',(1.11894887330541,-0.290879136862659,
0.107881990270302));
#13092=CARTESIAN_POINT('Ctrl Pts',(1.1160463456491,-0.279889827963178,0.133783682657561));
#13093=CARTESIAN_POINT('Ctrl Pts',(1.10909715583869,-0.251265615809407,
0.183354415742157));
#13094=CARTESIAN_POINT('Ctrl Pts',(1.10373487993589,-0.227269801620064,
0.212533521233765));
#13095=CARTESIAN_POINT('Ctrl Pts',(1.09443784939331,-0.177024326825049,
0.256354979351213));
#13096=CARTESIAN_POINT('Ctrl Pts',(1.08940878963422,-0.144299303100741,
0.276273267473431));
#13097=CARTESIAN_POINT('Ctrl Pts',(1.08431331394788,-0.0928409665394228,
0.2953917518996));
#13098=CARTESIAN_POINT('Ctrl Pts',(1.0830271513892,-0.0762225747374255,
0.300028012588062));
#13099=CARTESIAN_POINT('Ctrl Pts',(1.08212377959455,-0.0595300000000001,
0.303251606722892));
#13100=CARTESIAN_POINT('Origin',(0.,-0.05953,0.));
#13101=CARTESIAN_POINT('Origin',(0.,-0.05953,0.));
#13102=CARTESIAN_POINT('',(0.0589974094846122,-0.05953,1.07456964270265));
#13103=CARTESIAN_POINT('Origin',(0.,-0.05953,0.));
#13104=CARTESIAN_POINT('Origin',(-0.244773027351946,-0.05953,1.07242070340001));
#13105=CARTESIAN_POINT('Origin',(-0.244773027351946,0.,1.07242070340001));
#13106=CARTESIAN_POINT('',(-0.519393123750572,-0.05953,0.942555777842682));
#13107=CARTESIAN_POINT('Ctrl Pts',(-0.519393123750572,-0.05953,0.942555777842682));
#13108=CARTESIAN_POINT('Ctrl Pts',(-0.513714466572041,-0.0925528133349865,
0.945684988399766));
#13109=CARTESIAN_POINT('Ctrl Pts',(-0.503136848051455,-0.124911173756694,
0.951483858396181));
#13110=CARTESIAN_POINT('Ctrl Pts',(-0.47593627990192,-0.177924977804098,
0.965323333309091));
#13111=CARTESIAN_POINT('Ctrl Pts',(-0.460931856495794,-0.199697230012983,
0.972669835243841));
#13112=CARTESIAN_POINT('Ctrl Pts',(-0.426157505475872,-0.237895043532788,
0.988400002689705));
#13113=CARTESIAN_POINT('Ctrl Pts',(-0.406380688682952,-0.254319232363049,
0.996771768218699));
#13114=CARTESIAN_POINT('Ctrl Pts',(-0.364750145543744,-0.28018331644634,
1.01272583306292));
#13115=CARTESIAN_POINT('Ctrl Pts',(-0.340838910881557,-0.29104845371857,
1.02112815447116));
#13116=CARTESIAN_POINT('Ctrl Pts',(-0.290495481564827,-0.30527573347708,
1.036574285215));
#13117=CARTESIAN_POINT('Ctrl Pts',(-0.264056468041074,-0.308638795020976,
1.04359501395068));
#13118=CARTESIAN_POINT('Ctrl Pts',(-0.214892249704082,-0.308638795020976,
1.05481642595959));
#13119=CARTESIAN_POINT('Ctrl Pts',(-0.188025341585962,-0.30527573347708,
1.05996242598502));
#13120=CARTESIAN_POINT('Ctrl Pts',(-0.135965654106109,-0.29104845371857,
1.06788913840721));
#13121=CARTESIAN_POINT('Ctrl Pts',(-0.110776745452494,-0.28018331644634,
1.07069360430242));
#13122=CARTESIAN_POINT('Ctrl Pts',(-0.0663467128214646,-0.254319232363049,
1.07438230428002));
#13123=CARTESIAN_POINT('Ctrl Pts',(-0.0448960436540983,-0.237895043532788,
1.07542044338697));
#13124=CARTESIAN_POINT('Ctrl Pts',(-0.00674037211528124,-0.199697230012983,
1.07633607767727));
#13125=CARTESIAN_POINT('Ctrl Pts',(0.00996567398334777,-0.177924977804098,
1.07622728347683));
#13126=CARTESIAN_POINT('Ctrl Pts',(0.0404772621979741,-0.124911173756694,
1.07556023164702));
#13127=CARTESIAN_POINT('Ctrl Pts',(0.0525234025782719,-0.0925528133349865,
1.07492508698591));
#13128=CARTESIAN_POINT('Ctrl Pts',(0.0589974094846124,-0.05953,1.07456964270265));
#13129=CARTESIAN_POINT('Origin',(-0.244773027351946,-0.05953,1.07242070340001));
#13130=CARTESIAN_POINT('Origin',(0.,-0.05953,0.));
#13131=CARTESIAN_POINT('',(-0.803348093619616,-0.05953,0.716109245731214));
#13132=CARTESIAN_POINT('Origin',(0.,-0.05953,0.));
#13133=CARTESIAN_POINT('Origin',(-0.991065754692661,-0.05953,0.477272113029314));
#13134=CARTESIAN_POINT('Origin',(-0.991065754692661,0.,0.477272113029314));
#13135=CARTESIAN_POINT('',(-1.06075609691358,-0.05953,0.181596019242328));
#13136=CARTESIAN_POINT('Ctrl Pts',(-1.06075609691358,-0.05953,0.181596019242328));
#13137=CARTESIAN_POINT('Ctrl Pts',(-1.05966202740332,-0.0925528133349865,
0.187986803072856));
#13138=CARTESIAN_POINT('Ctrl Pts',(-1.05760072925372,-0.124911173756694,
0.199872254546857));
#13139=CARTESIAN_POINT('Ctrl Pts',(-1.05146158959546,-0.177924977804098,
0.22976728653846));
#13140=CARTESIAN_POINT('Ctrl Pts',(-1.04785021111757,-0.199697230012983,
0.246078686169301));
#13141=CARTESIAN_POINT('Ctrl Pts',(-1.03846709802406,-0.237895043532788,
0.283073967563097));
#13142=CARTESIAN_POINT('Ctrl Pts',(-1.03268176429485,-0.254319232363049,
0.303755815985685));
#13143=CARTESIAN_POINT('Ctrl Pts',(-1.01919893537026,-0.28018331644634,
0.346251081972725));
#13144=CARTESIAN_POINT('Ctrl Pts',(-1.01085972381132,-0.29104845371857,
0.370184399726282));
#13145=CARTESIAN_POINT('Ctrl Pts',(-0.99154738033959,-0.30527573347708,
0.419174982698463));
#13146=CARTESIAN_POINT('Ctrl Pts',(-0.980551951791748,-0.308638795020976,
0.444223188605045));
#13147=CARTESIAN_POINT('Ctrl Pts',(-0.958671816228589,-0.308638795020976,
0.489657758261848));
#13148=CARTESIAN_POINT('Ctrl Pts',(-0.945943877838127,-0.30527573347708,
0.51387163140139));
#13149=CARTESIAN_POINT('Ctrl Pts',(-0.91968254693063,-0.29104845371857,
0.559515758398093));
#13150=CARTESIAN_POINT('Ctrl Pts',(-0.906170138993533,-0.28018331644634,
0.580957796077825));
#13151=CARTESIAN_POINT('Ctrl Pts',(-0.8813524085237,-0.254319232363049,
0.617994461173994));
#13152=CARTESIAN_POINT('Ctrl Pts',(-0.868789784891799,-0.237895043532788,
0.635412538795143));
#13153=CARTESIAN_POINT('Ctrl Pts',(-0.845715984518854,-0.199697230012983,
0.66581473268113));
#13154=CARTESIAN_POINT('Ctrl Pts',(-0.835214876415962,-0.177924977804098,
0.678808213394124));
#13155=CARTESIAN_POINT('Ctrl Pts',(-0.815669690204649,-0.124911173756694,
0.702247233627224));
#13156=CARTESIAN_POINT('Ctrl Pts',(-0.807662468433796,-0.0925528133349865,
0.711269279199861));
#13157=CARTESIAN_POINT('Ctrl Pts',(-0.803348093619616,-0.05953,0.716109245731214));
#13158=CARTESIAN_POINT('Origin',(-0.991065754692661,-0.05953,0.477272113029314));
#13159=CARTESIAN_POINT('Origin',(0.,-0.05953,0.));
#13160=CARTESIAN_POINT('',(-1.076188,-0.05953,1.31795018948079E-16));
#13161=CARTESIAN_POINT('Origin',(0.,-0.05953,0.));
#13162=CARTESIAN_POINT('',(-1.06075609691358,-0.05953,-0.181596019242328));
#13163=CARTESIAN_POINT('Origin',(0.,-0.05953,0.));
#13164=CARTESIAN_POINT('Origin',(-0.991065754692661,-0.05953,-0.477272113029314));
#13165=CARTESIAN_POINT('Origin',(-0.991065754692661,0.,-0.477272113029314));
#13166=CARTESIAN_POINT('',(-0.803348093619616,-0.05953,-0.716109245731215));
#13167=CARTESIAN_POINT('Ctrl Pts',(-0.803348093619616,-0.05953,-0.716109245731215));
#13168=CARTESIAN_POINT('Ctrl Pts',(-0.807662468433795,-0.0925528133349865,
-0.711269279199862));
#13169=CARTESIAN_POINT('Ctrl Pts',(-0.815669690204649,-0.124911173756694,
-0.702247233627224));
#13170=CARTESIAN_POINT('Ctrl Pts',(-0.835214876415962,-0.177924977804098,
-0.678808213394124));
#13171=CARTESIAN_POINT('Ctrl Pts',(-0.845715984518854,-0.199697230012983,
-0.66581473268113));
#13172=CARTESIAN_POINT('Ctrl Pts',(-0.868789784891799,-0.237895043532788,
-0.635412538795143));
#13173=CARTESIAN_POINT('Ctrl Pts',(-0.8813524085237,-0.254319232363049,
-0.617994461173994));
#13174=CARTESIAN_POINT('Ctrl Pts',(-0.906170138993533,-0.28018331644634,
-0.580957796077826));
#13175=CARTESIAN_POINT('Ctrl Pts',(-0.91968254693063,-0.29104845371857,
-0.559515758398093));
#13176=CARTESIAN_POINT('Ctrl Pts',(-0.945943877838127,-0.30527573347708,
-0.51387163140139));
#13177=CARTESIAN_POINT('Ctrl Pts',(-0.958671816228589,-0.308638795020976,
-0.489657758261848));
#13178=CARTESIAN_POINT('Ctrl Pts',(-0.980551951791748,-0.308638795020976,
-0.444223188605045));
#13179=CARTESIAN_POINT('Ctrl Pts',(-0.99154738033959,-0.30527573347708,
-0.419174982698463));
#13180=CARTESIAN_POINT('Ctrl Pts',(-1.01085972381132,-0.29104845371857,
-0.370184399726282));
#13181=CARTESIAN_POINT('Ctrl Pts',(-1.01919893537026,-0.28018331644634,
-0.346251081972725));
#13182=CARTESIAN_POINT('Ctrl Pts',(-1.03268176429485,-0.254319232363049,
-0.303755815985685));
#13183=CARTESIAN_POINT('Ctrl Pts',(-1.03846709802406,-0.237895043532788,
-0.283073967563097));
#13184=CARTESIAN_POINT('Ctrl Pts',(-1.04785021111757,-0.199697230012983,
-0.246078686169302));
#13185=CARTESIAN_POINT('Ctrl Pts',(-1.05146158959546,-0.177924977804098,
-0.229767286538461));
#13186=CARTESIAN_POINT('Ctrl Pts',(-1.05760072925372,-0.124911173756694,
-0.199872254546858));
#13187=CARTESIAN_POINT('Ctrl Pts',(-1.05966202740332,-0.0925528133349864,
-0.187986803072857));
#13188=CARTESIAN_POINT('Ctrl Pts',(-1.06075609691358,-0.05953,-0.181596019242328));
#13189=CARTESIAN_POINT('Origin',(-0.991065754692661,-0.05953,-0.477272113029314));
#13190=CARTESIAN_POINT('Origin',(0.,-0.05953,0.));
#13191=CARTESIAN_POINT('',(-0.519393123750572,-0.05953,-0.942555777842682));
#13192=CARTESIAN_POINT('Origin',(0.,-0.05953,0.));
#13193=CARTESIAN_POINT('Origin',(-0.244773027351946,-0.05953,-1.07242070340001));
#13194=CARTESIAN_POINT('Origin',(-0.244773027351946,0.,-1.07242070340001));
#13195=CARTESIAN_POINT('',(0.0589974094846125,-0.05953,-1.07456964270265));
#13196=CARTESIAN_POINT('Ctrl Pts',(0.0589974094846127,-0.05953,-1.07456964270265));
#13197=CARTESIAN_POINT('Ctrl Pts',(0.0525234025782722,-0.0925528133349865,
-1.07492508698591));
#13198=CARTESIAN_POINT('Ctrl Pts',(0.0404772621979744,-0.124911173756694,
-1.07556023164702));
#13199=CARTESIAN_POINT('Ctrl Pts',(0.0099656739833481,-0.177924977804098,
-1.07622728347683));
#13200=CARTESIAN_POINT('Ctrl Pts',(-0.00674037211528096,-0.199697230012983,
-1.07633607767727));
#13201=CARTESIAN_POINT('Ctrl Pts',(-0.044896043654098,-0.237895043532788,
-1.07542044338697));
#13202=CARTESIAN_POINT('Ctrl Pts',(-0.0663467128214644,-0.254319232363049,
-1.07438230428002));
#13203=CARTESIAN_POINT('Ctrl Pts',(-0.110776745452493,-0.28018331644634,
-1.07069360430242));
#13204=CARTESIAN_POINT('Ctrl Pts',(-0.135965654106109,-0.29104845371857,
-1.06788913840721));
#13205=CARTESIAN_POINT('Ctrl Pts',(-0.188025341585962,-0.30527573347708,
-1.05996242598502));
#13206=CARTESIAN_POINT('Ctrl Pts',(-0.214892249704082,-0.308638795020976,
-1.05481642595959));
#13207=CARTESIAN_POINT('Ctrl Pts',(-0.264056468041074,-0.308638795020976,
-1.04359501395068));
#13208=CARTESIAN_POINT('Ctrl Pts',(-0.290495481564827,-0.30527573347708,
-1.036574285215));
#13209=CARTESIAN_POINT('Ctrl Pts',(-0.340838910881557,-0.291048453718569,
-1.02112815447116));
#13210=CARTESIAN_POINT('Ctrl Pts',(-0.364750145543744,-0.28018331644634,
-1.01272583306292));
#13211=CARTESIAN_POINT('Ctrl Pts',(-0.406380688682952,-0.254319232363049,
-0.996771768218699));
#13212=CARTESIAN_POINT('Ctrl Pts',(-0.426157505475872,-0.237895043532788,
-0.988400002689705));
#13213=CARTESIAN_POINT('Ctrl Pts',(-0.460931856495794,-0.199697230012983,
-0.972669835243841));
#13214=CARTESIAN_POINT('Ctrl Pts',(-0.475936279901919,-0.177924977804098,
-0.965323333309091));
#13215=CARTESIAN_POINT('Ctrl Pts',(-0.503136848051454,-0.124911173756694,
-0.951483858396181));
#13216=CARTESIAN_POINT('Ctrl Pts',(-0.513714466572041,-0.0925528133349865,
-0.945684988399766));
#13217=CARTESIAN_POINT('Ctrl Pts',(-0.519393123750572,-0.05953,-0.942555777842682));
#13218=CARTESIAN_POINT('Origin',(-0.244773027351946,-0.05953,-1.07242070340001));
#13219=CARTESIAN_POINT('Origin',(0.,-0.05953,0.));
#13220=CARTESIAN_POINT('',(0.413083465285518,-0.05953,-0.993751811093549));
#13221=CARTESIAN_POINT('Origin',(0.,-0.05953,0.));
#13222=CARTESIAN_POINT('Origin',(0.685838782044607,-0.05953,-0.860014630714833));
#13223=CARTESIAN_POINT('Origin',(0.685838782044607,0.,-0.860014630714833));
#13224=CARTESIAN_POINT('',(0.876916659919095,-0.05953,-0.623857181492959));
#13225=CARTESIAN_POINT('Ctrl Pts',(0.876916659919095,-0.05953,-0.623857181492958));
#13226=CARTESIAN_POINT('Ctrl Pts',(0.873158080166742,-0.0925528133349865,
-0.62914037979579));
#13227=CARTESIAN_POINT('Ctrl Pts',(0.866144010579847,-0.124911173756694,
-0.638954437806245));
#13228=CARTESIAN_POINT('Ctrl Pts',(0.847641868610495,-0.177924977804098,
-0.663225258065736));
#13229=CARTESIAN_POINT('Ctrl Pts',(0.837310877969633,-0.199697230012983,
-0.676354402927683));
#13230=CARTESIAN_POINT('Ctrl Pts',(0.81280533416753,-0.237895043532788,
-0.705614819529209));
#13231=CARTESIAN_POINT('Ctrl Pts',(0.798619410861634,-0.254319232363049,
-0.721738358858166));
#13232=CARTESIAN_POINT('Ctrl Pts',(0.768033796848072,-0.28018331644634,
-0.754175290318038));
#13233=CARTESIAN_POINT('Ctrl Pts',(0.750136149454208,-0.29104845371857,
-0.772120216227122));
#13234=CARTESIAN_POINT('Ctrl Pts',(0.711480111898423,-0.30527573347708,
-0.807879894508811));
#13235=CARTESIAN_POINT('Ctrl Pts',(0.690705563850638,-0.308638795020976,
-0.825676810575913));
#13236=CARTESIAN_POINT('Ctrl Pts',(0.651278921914856,-0.308638795020976,
-0.857118508332695));
#13237=CARTESIAN_POINT('Ctrl Pts',(0.629305439856167,-0.30527573347708,
-0.873412008702649));
#13238=CARTESIAN_POINT('Ctrl Pts',(0.585840553788742,-0.29104845371857,
-0.903141581680914));
#13239=CARTESIAN_POINT('Ctrl Pts',(0.564362943424239,-0.28018331644634,
-0.916597376014514));
#13240=CARTESIAN_POINT('Ctrl Pts',(0.525933334162556,-0.254319232363049,
-0.939198248544427));
#13241=CARTESIAN_POINT('Ctrl Pts',(0.507057380724533,-0.237895043532788,
-0.949440676105255));
#13242=CARTESIAN_POINT('Ctrl Pts',(0.473077587363686,-0.199697230012983,
-0.966820759530997));
#13243=CARTESIAN_POINT('Ctrl Pts',(0.457978755888596,-0.177924977804098,
-0.973971221090534));
#13244=CARTESIAN_POINT('Ctrl Pts',(0.430199341854858,-0.124911173756694,
-0.986608710139579));
#13245=CARTESIAN_POINT('Ctrl Pts',(0.419070565453384,-0.0925528133349865,
-0.991263089003441));
#13246=CARTESIAN_POINT('Ctrl Pts',(0.413083465285518,-0.05953,-0.993751811093549));
#13247=CARTESIAN_POINT('Origin',(0.685838782044607,-0.05953,-0.860014630714833));
#13248=CARTESIAN_POINT('Origin',(0.,-0.208355,0.));
#13249=CARTESIAN_POINT('',(-1.076188,-0.35718,1.31795018948079E-16));
#13250=CARTESIAN_POINT('Origin',(0.,-0.35718,0.));
#13251=CARTESIAN_POINT('',(-1.076188,-0.208355,1.31795018948079E-16));
#13252=CARTESIAN_POINT('',(1.03449977959455,-0.05953,0.296632461748266));
#13253=CARTESIAN_POINT('Origin',(0.,-0.05953,0.));
#13254=CARTESIAN_POINT('',(1.03449977959455,-0.05953,-0.296632461748266));
#13255=CARTESIAN_POINT('Ctrl Pts',(1.03449977959455,-0.05953,0.296632461748267));
#13256=CARTESIAN_POINT('Ctrl Pts',(1.03628691421076,-0.0925528133349865,
0.290399865505497));
#13257=CARTESIAN_POINT('Ctrl Pts',(1.03958665287714,-0.124911173756694,
0.278797079997872));
#13258=CARTESIAN_POINT('Ctrl Pts',(1.0470264474309,-0.177924977804098,0.249198913998601));
#13259=CARTESIAN_POINT('Ctrl Pts',(1.05084995891418,-0.199697230012983,
0.232935932341942));
#13260=CARTESIAN_POINT('Ctrl Pts',(1.05844771715377,-0.237895043532788,
0.195533155353269));
#13261=CARTESIAN_POINT('Ctrl Pts',(1.06220882929878,-0.254319232363049,
0.17438929156337));
#13262=CARTESIAN_POINT('Ctrl Pts',(1.06849922508772,-0.28018331644634,0.130252399648131));
#13263=CARTESIAN_POINT('Ctrl Pts',(1.07137013248666,-0.29104845371857,0.105070977154072));
#13264=CARTESIAN_POINT('Ctrl Pts',(1.07522652957392,-0.30527573347708,0.0525526752791107));
#13265=CARTESIAN_POINT('Ctrl Pts',(1.076188,-0.308638795020976,0.025214283908933));
#13266=CARTESIAN_POINT('Ctrl Pts',(1.076188,-0.308638795020976,-0.025214283908933));
#13267=CARTESIAN_POINT('Ctrl Pts',(1.07522652957392,-0.30527573347708,-0.0525526752791107));
#13268=CARTESIAN_POINT('Ctrl Pts',(1.07137013248666,-0.29104845371857,-0.105070977154072));
#13269=CARTESIAN_POINT('Ctrl Pts',(1.06849922508772,-0.28018331644634,-0.130252399648131));
#13270=CARTESIAN_POINT('Ctrl Pts',(1.06220882929878,-0.254319232363049,
-0.17438929156337));
#13271=CARTESIAN_POINT('Ctrl Pts',(1.05844771715377,-0.237895043532788,
-0.195533155353269));
#13272=CARTESIAN_POINT('Ctrl Pts',(1.05084995891418,-0.199697230012983,
-0.232935932341942));
#13273=CARTESIAN_POINT('Ctrl Pts',(1.0470264474309,-0.177924977804098,-0.249198913998601));
#13274=CARTESIAN_POINT('Ctrl Pts',(1.03958665287714,-0.124911173756694,
-0.278797079997872));
#13275=CARTESIAN_POINT('Ctrl Pts',(1.03628691421076,-0.0925528133349865,
-0.290399865505497));
#13276=CARTESIAN_POINT('Ctrl Pts',(1.03449977959455,-0.05953,-0.296632461748267));
#13277=CARTESIAN_POINT('Origin',(0.,-0.05953,0.));
#13278=CARTESIAN_POINT('Origin',(0.,-0.05953,0.));
#13279=CARTESIAN_POINT('Origin',(1.1,-0.05953,0.));
#13280=CARTESIAN_POINT('Origin',(1.1,0.,0.));
#13281=CARTESIAN_POINT('Origin',(1.1,-0.05953,0.));
#13282=CARTESIAN_POINT('Origin',(0.,-0.35718,0.));
#13283=CARTESIAN_POINT('Origin',(0.,-0.05953,0.));
#14755=UNCERTAINTY_MEASURE_WITH_UNIT(LENGTH_MEASURE(0.001),#14823,
'DISTANCE_ACCURACY_VALUE',
'Maximum model space distance between geometric entities at asserted c
onnectivities');
#14777=UNCERTAINTY_MEASURE_WITH_UNIT(LENGTH_MEASURE(0.001),#14823,
'DISTANCE_ACCURACY_VALUE',
'Maximum model space distance between geometric entities at asserted c
onnectivities');
#14800=(
GEOMETRIC_REPRESENTATION_CONTEXT(3)
GLOBAL_UNCERTAINTY_ASSIGNED_CONTEXT((#14755))
GLOBAL_UNIT_ASSIGNED_CONTEXT((#14823,#14825,#14826))
REPRESENTATION_CONTEXT('','3D')
);
#14822=(
GEOMETRIC_REPRESENTATION_CONTEXT(3)
GLOBAL_UNCERTAINTY_ASSIGNED_CONTEXT((#14777))
GLOBAL_UNIT_ASSIGNED_CONTEXT((#14823,#14825,#14826))
REPRESENTATION_CONTEXT('','3D')
);
#14823=(
LENGTH_UNIT()
NAMED_UNIT(*)
SI_UNIT(.CENTI.,.METRE.)
);
#14825=(
NAMED_UNIT(*)
PLANE_ANGLE_UNIT()
SI_UNIT($,.RADIAN.)
);
#14826=(
NAMED_UNIT(*)
SI_UNIT($,.STERADIAN.)
SOLID_ANGLE_UNIT()
);
#14849=SHAPE_DEFINITION_REPRESENTATION(#14893,#15020);
#14893=PRODUCT_DEFINITION_SHAPE('',$,#15065);
#15020=SHAPE_REPRESENTATION('',(#8678),#14800);
#15042=PRODUCT_DEFINITION_CONTEXT('part definition',#15176,'design');
#15065=PRODUCT_DEFINITION('Cage','Cage',#15109,#15042);
#15109=PRODUCT_DEFINITION_FORMATION('',$,#15200);
#15176=APPLICATION_CONTEXT(
'Core Data for Automotive Mechanical Design Process');
#15177=PRODUCT_CONTEXT('part definition',#15176,'mechanical');
#15200=PRODUCT('Cage','Cage','Cage',(#15177));
#15278=COLOUR_RGB('Grey',0.48,0.52,0.57);
#15279=FILL_AREA_STYLE_COLOUR('',#15278);
#15280=FILL_AREA_STYLE('',(#15279));
#15281=SURFACE_STYLE_FILL_AREA(#15280);
#15282=SURFACE_SIDE_STYLE('',(#15281));
#15283=SURFACE_STYLE_USAGE(.BOTH.,#15282);
#15284=PRESENTATION_STYLE_ASSIGNMENT((#15283));
ENDSEC;
END-ISO-10303-21;
